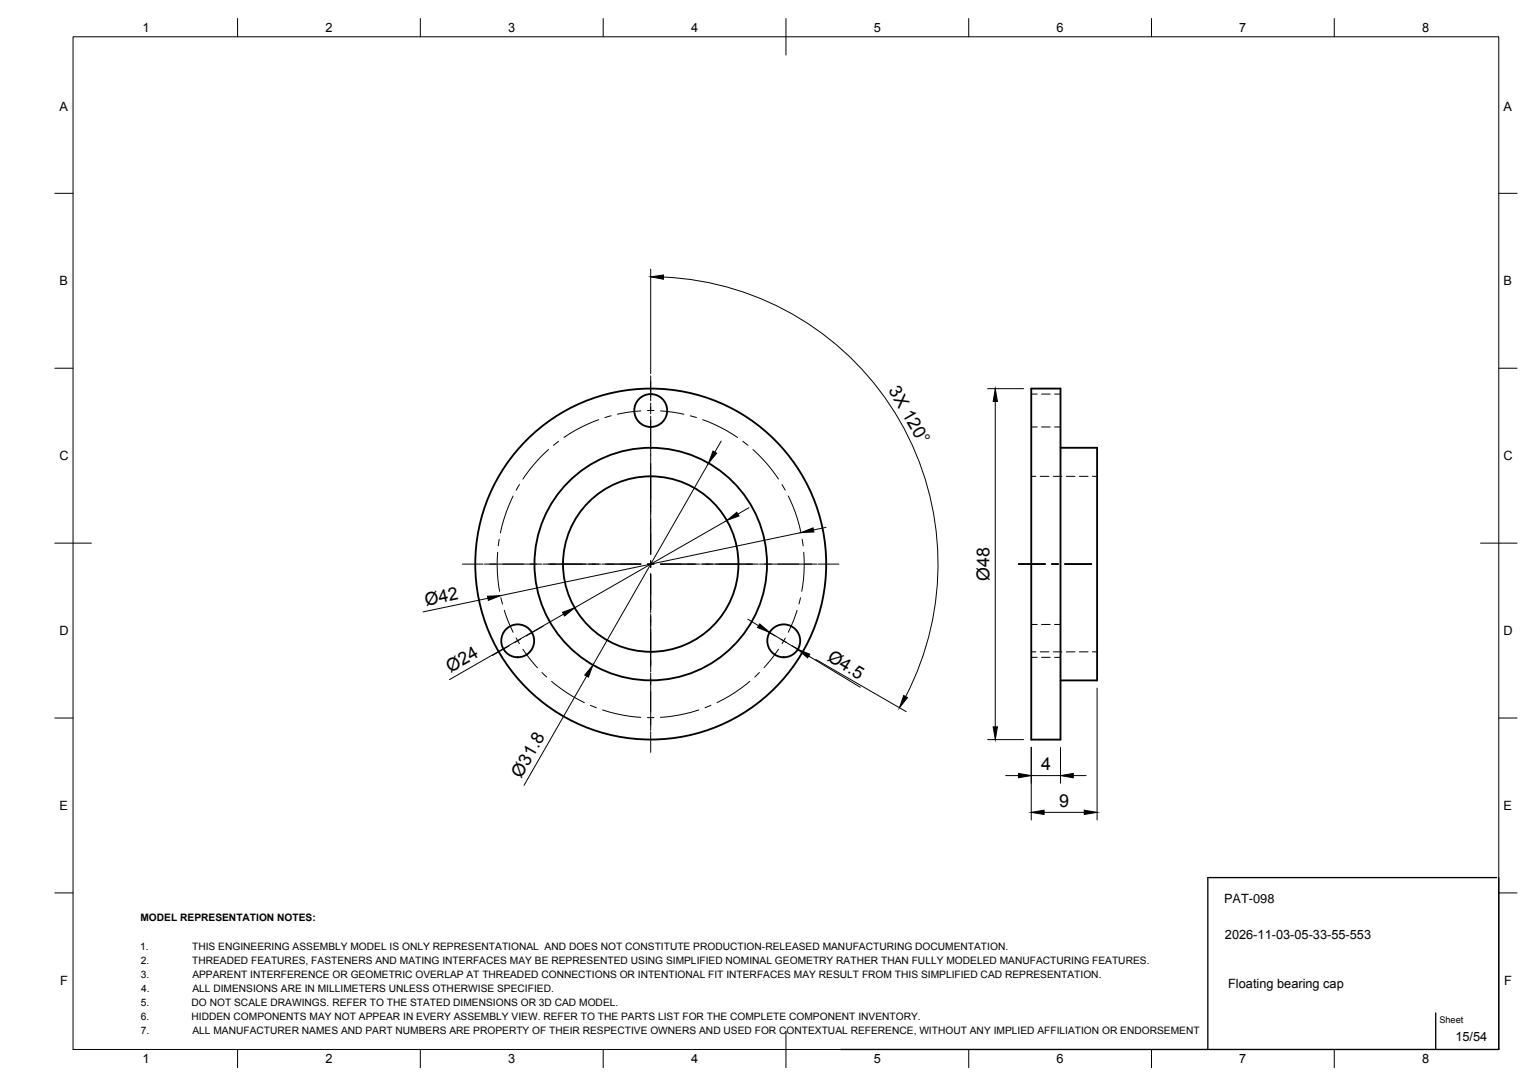
ISO-10303-21;
HEADER;
/* Generated by software containing ST-Developer
 * from STEP Tools, Inc. (www.steptools.com) 
 */

FILE_DESCRIPTION(
/* description */ ('Spring compression tester'),
/* implementation_level */ '2;1');

FILE_NAME(
/* name */ 'Floating bearing cap.step',
/* time_stamp */ '2026-10-28T03:24:11-07:00',
/* author */ (''),
/* organization */ (''),
/* preprocessor_version */ 'ST-DEVELOPER v20.2',
/* originating_system */ 'Autodesk Translation Framework v15.17.0.0',
/* authorisation */ '');

FILE_SCHEMA (('AUTOMOTIVE_DESIGN { 1 0 10303 214 3 1 1 }'));
ENDSEC;

DATA;
#10=MECHANICAL_DESIGN_GEOMETRIC_PRESENTATION_REPRESENTATION('',(#1116),#43521);
#996=SHAPE_REPRESENTATION_RELATIONSHIP('SRR','None',#43808,#1056);
#1056=ADVANCED_BREP_SHAPE_REPRESENTATION('',(#1191),#43468);
#1116=STYLED_ITEM('',(#44202),#1191);
#1191=MANIFOLD_SOLID_BREP('Body1',#18553);
#1376=FACE_BOUND('',#3547,.T.);
#1377=FACE_BOUND('',#3551,.T.);
#1378=FACE_BOUND('',#3552,.T.);
#1379=FACE_BOUND('',#3553,.T.);
#1380=FACE_BOUND('',#3554,.T.);
#1381=FACE_BOUND('',#3556,.T.);
#1382=FACE_BOUND('',#3557,.T.);
#1383=FACE_BOUND('',#3558,.T.);
#1384=FACE_BOUND('',#3559,.T.);
#1704=PLANE('',#19677);
#1705=PLANE('',#19684);
#1706=PLANE('',#19685);
#2366=FACE_OUTER_BOUND('',#3542,.T.);
#2367=FACE_OUTER_BOUND('',#3543,.T.);
#2368=FACE_OUTER_BOUND('',#3544,.T.);
#2369=FACE_OUTER_BOUND('',#3545,.T.);
#2370=FACE_OUTER_BOUND('',#3546,.T.);
#2371=FACE_OUTER_BOUND('',#3548,.T.);
#2372=FACE_OUTER_BOUND('',#3549,.T.);
#2373=FACE_OUTER_BOUND('',#3550,.T.);
#2374=FACE_OUTER_BOUND('',#3555,.T.);
#3542=EDGE_LOOP('',(#13111,#13112,#13113,#13114));
#3543=EDGE_LOOP('',(#13115,#13116,#13117,#13118));
#3544=EDGE_LOOP('',(#13119,#13120,#13121,#13122));
#3545=EDGE_LOOP('',(#13123,#13124,#13125,#13126));
#3546=EDGE_LOOP('',(#13127));
#3547=EDGE_LOOP('',(#13128));
#3548=EDGE_LOOP('',(#13129,#13130,#13131,#13132));
#3549=EDGE_LOOP('',(#13133,#13134,#13135,#13136));
#3550=EDGE_LOOP('',(#13137));
#3551=EDGE_LOOP('',(#13138));
#3552=EDGE_LOOP('',(#13139));
#3553=EDGE_LOOP('',(#13140));
#3554=EDGE_LOOP('',(#13141));
#3555=EDGE_LOOP('',(#13142));
#3556=EDGE_LOOP('',(#13143));
#3557=EDGE_LOOP('',(#13144));
#3558=EDGE_LOOP('',(#13145));
#3559=EDGE_LOOP('',(#13146));
#4883=LINE('',#27412,#6315);
#4884=LINE('',#27418,#6316);
#4885=LINE('',#27424,#6317);
#4886=LINE('',#27430,#6318);
#4887=LINE('',#27437,#6319);
#4888=LINE('',#27443,#6320);
#6315=VECTOR('',#22239,0.225);
#6316=VECTOR('',#22246,0.225);
#6317=VECTOR('',#22253,0.225);
#6318=VECTOR('',#22260,1.59);
#6319=VECTOR('',#22269,1.2);
#6320=VECTOR('',#22276,2.4);
#7640=CIRCLE('',#19666,0.225);
#7641=CIRCLE('',#19667,0.225);
#7642=CIRCLE('',#19669,0.225);
#7643=CIRCLE('',#19670,0.225);
#7644=CIRCLE('',#19672,0.225);
#7645=CIRCLE('',#19673,0.225);
#7646=CIRCLE('',#19675,1.59);
#7647=CIRCLE('',#19676,1.59);
#7648=CIRCLE('',#19678,1.2);
#7649=CIRCLE('',#19680,1.2);
#7650=CIRCLE('',#19682,2.4);
#7651=CIRCLE('',#19683,2.4);
#8434=VERTEX_POINT('',#27409);
#8435=VERTEX_POINT('',#27411);
#8436=VERTEX_POINT('',#27415);
#8437=VERTEX_POINT('',#27417);
#8438=VERTEX_POINT('',#27421);
#8439=VERTEX_POINT('',#27423);
#8440=VERTEX_POINT('',#27427);
#8441=VERTEX_POINT('',#27429);
#8442=VERTEX_POINT('',#27433);
#8443=VERTEX_POINT('',#27436);
#8444=VERTEX_POINT('',#27440);
#8445=VERTEX_POINT('',#27442);
#10220=EDGE_CURVE('',#8434,#8434,#7640,.T.);
#10221=EDGE_CURVE('',#8434,#8435,#4883,.T.);
#10222=EDGE_CURVE('',#8435,#8435,#7641,.T.);
#10223=EDGE_CURVE('',#8436,#8436,#7642,.T.);
#10224=EDGE_CURVE('',#8436,#8437,#4884,.T.);
#10225=EDGE_CURVE('',#8437,#8437,#7643,.T.);
#10226=EDGE_CURVE('',#8438,#8438,#7644,.T.);
#10227=EDGE_CURVE('',#8438,#8439,#4885,.T.);
#10228=EDGE_CURVE('',#8439,#8439,#7645,.T.);
#10229=EDGE_CURVE('',#8440,#8440,#7646,.T.);
#10230=EDGE_CURVE('',#8440,#8441,#4886,.T.);
#10231=EDGE_CURVE('',#8441,#8441,#7647,.T.);
#10232=EDGE_CURVE('',#8442,#8442,#7648,.T.);
#10233=EDGE_CURVE('',#8442,#8443,#4887,.T.);
#10234=EDGE_CURVE('',#8443,#8443,#7649,.T.);
#10235=EDGE_CURVE('',#8444,#8444,#7650,.T.);
#10236=EDGE_CURVE('',#8444,#8445,#4888,.T.);
#10237=EDGE_CURVE('',#8445,#8445,#7651,.T.);
#13111=ORIENTED_EDGE('',*,*,#10220,.F.);
#13112=ORIENTED_EDGE('',*,*,#10221,.T.);
#13113=ORIENTED_EDGE('',*,*,#10222,.F.);
#13114=ORIENTED_EDGE('',*,*,#10221,.F.);
#13115=ORIENTED_EDGE('',*,*,#10223,.F.);
#13116=ORIENTED_EDGE('',*,*,#10224,.T.);
#13117=ORIENTED_EDGE('',*,*,#10225,.F.);
#13118=ORIENTED_EDGE('',*,*,#10224,.F.);
#13119=ORIENTED_EDGE('',*,*,#10226,.F.);
#13120=ORIENTED_EDGE('',*,*,#10227,.T.);
#13121=ORIENTED_EDGE('',*,*,#10228,.F.);
#13122=ORIENTED_EDGE('',*,*,#10227,.F.);
#13123=ORIENTED_EDGE('',*,*,#10229,.F.);
#13124=ORIENTED_EDGE('',*,*,#10230,.T.);
#13125=ORIENTED_EDGE('',*,*,#10231,.F.);
#13126=ORIENTED_EDGE('',*,*,#10230,.F.);
#13127=ORIENTED_EDGE('',*,*,#10229,.T.);
#13128=ORIENTED_EDGE('',*,*,#10232,.T.);
#13129=ORIENTED_EDGE('',*,*,#10232,.F.);
#13130=ORIENTED_EDGE('',*,*,#10233,.T.);
#13131=ORIENTED_EDGE('',*,*,#10234,.T.);
#13132=ORIENTED_EDGE('',*,*,#10233,.F.);
#13133=ORIENTED_EDGE('',*,*,#10235,.F.);
#13134=ORIENTED_EDGE('',*,*,#10236,.T.);
#13135=ORIENTED_EDGE('',*,*,#10237,.T.);
#13136=ORIENTED_EDGE('',*,*,#10236,.F.);
#13137=ORIENTED_EDGE('',*,*,#10235,.T.);
#13138=ORIENTED_EDGE('',*,*,#10222,.T.);
#13139=ORIENTED_EDGE('',*,*,#10225,.T.);
#13140=ORIENTED_EDGE('',*,*,#10228,.T.);
#13141=ORIENTED_EDGE('',*,*,#10231,.T.);
#13142=ORIENTED_EDGE('',*,*,#10237,.F.);
#13143=ORIENTED_EDGE('',*,*,#10220,.T.);
#13144=ORIENTED_EDGE('',*,*,#10223,.T.);
#13145=ORIENTED_EDGE('',*,*,#10226,.T.);
#13146=ORIENTED_EDGE('',*,*,#10234,.F.);
#17186=CYLINDRICAL_SURFACE('',#19665,0.225);
#17187=CYLINDRICAL_SURFACE('',#19668,0.225);
#17188=CYLINDRICAL_SURFACE('',#19671,0.225);
#17189=CYLINDRICAL_SURFACE('',#19674,1.59);
#17190=CYLINDRICAL_SURFACE('',#19679,1.2);
#17191=CYLINDRICAL_SURFACE('',#19681,2.4);
#17690=ADVANCED_FACE('',(#2366),#17186,.F.);
#17691=ADVANCED_FACE('',(#2367),#17187,.F.);
#17692=ADVANCED_FACE('',(#2368),#17188,.F.);
#17693=ADVANCED_FACE('',(#2369),#17189,.T.);
#17694=ADVANCED_FACE('',(#2370,#1376),#1704,.T.);
#17695=ADVANCED_FACE('',(#2371),#17190,.F.);
#17696=ADVANCED_FACE('',(#2372),#17191,.T.);
#17697=ADVANCED_FACE('',(#2373,#1377,#1378,#1379,#1380),#1705,.T.);
#17698=ADVANCED_FACE('',(#2374,#1381,#1382,#1383,#1384),#1706,.F.);
#18553=CLOSED_SHELL('',(#17690,#17691,#17692,#17693,#17694,#17695,#17696,
#17697,#17698));
#19664=AXIS2_PLACEMENT_3D('',#27407,#22233,#22234);
#19665=AXIS2_PLACEMENT_3D('',#27408,#22235,#22236);
#19666=AXIS2_PLACEMENT_3D('',#27410,#22237,#22238);
#19667=AXIS2_PLACEMENT_3D('',#27413,#22240,#22241);
#19668=AXIS2_PLACEMENT_3D('',#27414,#22242,#22243);
#19669=AXIS2_PLACEMENT_3D('',#27416,#22244,#22245);
#19670=AXIS2_PLACEMENT_3D('',#27419,#22247,#22248);
#19671=AXIS2_PLACEMENT_3D('',#27420,#22249,#22250);
#19672=AXIS2_PLACEMENT_3D('',#27422,#22251,#22252);
#19673=AXIS2_PLACEMENT_3D('',#27425,#22254,#22255);
#19674=AXIS2_PLACEMENT_3D('',#27426,#22256,#22257);
#19675=AXIS2_PLACEMENT_3D('',#27428,#22258,#22259);
#19676=AXIS2_PLACEMENT_3D('',#27431,#22261,#22262);
#19677=AXIS2_PLACEMENT_3D('',#27432,#22263,#22264);
#19678=AXIS2_PLACEMENT_3D('',#27434,#22265,#22266);
#19679=AXIS2_PLACEMENT_3D('',#27435,#22267,#22268);
#19680=AXIS2_PLACEMENT_3D('',#27438,#22270,#22271);
#19681=AXIS2_PLACEMENT_3D('',#27439,#22272,#22273);
#19682=AXIS2_PLACEMENT_3D('',#27441,#22274,#22275);
#19683=AXIS2_PLACEMENT_3D('',#27444,#22277,#22278);
#19684=AXIS2_PLACEMENT_3D('',#27445,#22279,#22280);
#19685=AXIS2_PLACEMENT_3D('',#27446,#22281,#22282);
#22233=DIRECTION('axis',(0.,0.,1.));
#22234=DIRECTION('refdir',(1.,0.,0.));
#22235=DIRECTION('center_axis',(0.,0.,1.));
#22236=DIRECTION('ref_axis',(1.,0.,0.));
#22237=DIRECTION('center_axis',(0.,0.,1.));
#22238=DIRECTION('ref_axis',(1.,0.,0.));
#22239=DIRECTION('',(0.,0.,1.));
#22240=DIRECTION('center_axis',(0.,0.,-1.));
#22241=DIRECTION('ref_axis',(1.,0.,0.));
#22242=DIRECTION('center_axis',(0.,0.,1.));
#22243=DIRECTION('ref_axis',(1.,0.,0.));
#22244=DIRECTION('center_axis',(0.,0.,1.));
#22245=DIRECTION('ref_axis',(1.,0.,0.));
#22246=DIRECTION('',(0.,0.,1.));
#22247=DIRECTION('center_axis',(0.,0.,-1.));
#22248=DIRECTION('ref_axis',(1.,0.,0.));
#22249=DIRECTION('center_axis',(0.,0.,1.));
#22250=DIRECTION('ref_axis',(1.,0.,0.));
#22251=DIRECTION('center_axis',(0.,0.,1.));
#22252=DIRECTION('ref_axis',(1.,0.,0.));
#22253=DIRECTION('',(0.,0.,1.));
#22254=DIRECTION('center_axis',(0.,0.,-1.));
#22255=DIRECTION('ref_axis',(1.,0.,0.));
#22256=DIRECTION('center_axis',(0.,0.,1.));
#22257=DIRECTION('ref_axis',(1.,0.,0.));
#22258=DIRECTION('center_axis',(0.,0.,1.));
#22259=DIRECTION('ref_axis',(1.,0.,0.));
#22260=DIRECTION('',(0.,0.,-1.));
#22261=DIRECTION('center_axis',(0.,0.,-1.));
#22262=DIRECTION('ref_axis',(1.,0.,0.));
#22263=DIRECTION('center_axis',(0.,0.,1.));
#22264=DIRECTION('ref_axis',(1.,0.,0.));
#22265=DIRECTION('center_axis',(0.,0.,-1.));
#22266=DIRECTION('ref_axis',(1.,0.,0.));
#22267=DIRECTION('center_axis',(0.,0.,1.));
#22268=DIRECTION('ref_axis',(1.,0.,0.));
#22269=DIRECTION('',(0.,0.,-1.));
#22270=DIRECTION('center_axis',(0.,0.,-1.));
#22271=DIRECTION('ref_axis',(1.,0.,0.));
#22272=DIRECTION('center_axis',(0.,0.,1.));
#22273=DIRECTION('ref_axis',(1.,0.,0.));
#22274=DIRECTION('center_axis',(0.,0.,1.));
#22275=DIRECTION('ref_axis',(1.,0.,0.));
#22276=DIRECTION('',(0.,0.,-1.));
#22277=DIRECTION('center_axis',(0.,0.,1.));
#22278=DIRECTION('ref_axis',(1.,0.,0.));
#22279=DIRECTION('center_axis',(0.,0.,1.));
#22280=DIRECTION('ref_axis',(1.,0.,0.));
#22281=DIRECTION('center_axis',(0.,0.,1.));
#22282=DIRECTION('ref_axis',(1.,0.,0.));
#27407=CARTESIAN_POINT('',(0.,0.,0.));
#27408=CARTESIAN_POINT('Origin',(2.1,5.,1.5));
#27409=CARTESIAN_POINT('',(1.875,5.,1.6));
#27410=CARTESIAN_POINT('Origin',(2.1,5.,1.6));
#27411=CARTESIAN_POINT('',(1.875,5.,2.));
#27412=CARTESIAN_POINT('',(1.875,5.,1.5));
#27413=CARTESIAN_POINT('Origin',(2.1,5.,2.));
#27414=CARTESIAN_POINT('Origin',(-1.05,6.81865334794732,1.5));
#27415=CARTESIAN_POINT('',(-1.275,6.81865334794732,1.6));
#27416=CARTESIAN_POINT('Origin',(-1.05,6.81865334794732,1.6));
#27417=CARTESIAN_POINT('',(-1.275,6.81865334794732,2.));
#27418=CARTESIAN_POINT('',(-1.275,6.81865334794732,1.5));
#27419=CARTESIAN_POINT('Origin',(-1.05,6.81865334794732,2.));
#27420=CARTESIAN_POINT('Origin',(-1.05,3.18134665205268,1.5));
#27421=CARTESIAN_POINT('',(-1.275,3.18134665205268,1.6));
#27422=CARTESIAN_POINT('Origin',(-1.05,3.18134665205268,1.6));
#27423=CARTESIAN_POINT('',(-1.275,3.18134665205268,2.));
#27424=CARTESIAN_POINT('',(-1.275,3.18134665205268,1.5));
#27425=CARTESIAN_POINT('Origin',(-1.05,3.18134665205268,2.));
#27426=CARTESIAN_POINT('Origin',(0.,5.,2.));
#27427=CARTESIAN_POINT('',(-1.59,5.,2.5));
#27428=CARTESIAN_POINT('Origin',(0.,5.,2.5));
#27429=CARTESIAN_POINT('',(-1.59,5.,2.));
#27430=CARTESIAN_POINT('',(-1.59,5.,2.));
#27431=CARTESIAN_POINT('Origin',(0.,5.,2.));
#27432=CARTESIAN_POINT('Origin',(0.,5.,2.5));
#27433=CARTESIAN_POINT('',(-1.2,5.,2.5));
#27434=CARTESIAN_POINT('Origin',(0.,5.,2.5));
#27435=CARTESIAN_POINT('Origin',(0.,5.,1.6));
#27436=CARTESIAN_POINT('',(-1.2,5.,1.6));
#27437=CARTESIAN_POINT('',(-1.2,5.,1.6));
#27438=CARTESIAN_POINT('Origin',(0.,5.,1.6));
#27439=CARTESIAN_POINT('Origin',(0.,5.,1.6));
#27440=CARTESIAN_POINT('',(-2.4,5.,2.));
#27441=CARTESIAN_POINT('Origin',(0.,5.,2.));
#27442=CARTESIAN_POINT('',(-2.4,5.,1.6));
#27443=CARTESIAN_POINT('',(-2.4,5.,1.6));
#27444=CARTESIAN_POINT('Origin',(0.,5.,1.6));
#27445=CARTESIAN_POINT('Origin',(0.,5.,2.));
#27446=CARTESIAN_POINT('Origin',(0.,5.,1.6));
#43400=UNCERTAINTY_MEASURE_WITH_UNIT(LENGTH_MEASURE(0.001),#43522,
'DISTANCE_ACCURACY_VALUE',
'Maximum model space distance between geometric entities at asserted c
onnectivities');
#43453=UNCERTAINTY_MEASURE_WITH_UNIT(LENGTH_MEASURE(0.001),#43522,
'DISTANCE_ACCURACY_VALUE',
'Maximum model space distance between geometric entities at asserted c
onnectivities');
#43468=(
GEOMETRIC_REPRESENTATION_CONTEXT(3)
GLOBAL_UNCERTAINTY_ASSIGNED_CONTEXT((#43400))
GLOBAL_UNIT_ASSIGNED_CONTEXT((#43522,#43524,#43525))
REPRESENTATION_CONTEXT('','3D')
);
#43521=(
GEOMETRIC_REPRESENTATION_CONTEXT(3)
GLOBAL_UNCERTAINTY_ASSIGNED_CONTEXT((#43453))
GLOBAL_UNIT_ASSIGNED_CONTEXT((#43522,#43524,#43525))
REPRESENTATION_CONTEXT('','3D')
);
#43522=(
LENGTH_UNIT()
NAMED_UNIT(*)
SI_UNIT(.CENTI.,.METRE.)
);
#43524=(
NAMED_UNIT(*)
PLANE_ANGLE_UNIT()
SI_UNIT($,.RADIAN.)
);
#43525=(
NAMED_UNIT(*)
SI_UNIT($,.STERADIAN.)
SOLID_ANGLE_UNIT()
);
#43540=SHAPE_DEFINITION_REPRESENTATION(#43607,#43808);
#43607=PRODUCT_DEFINITION_SHAPE('',$,#43876);
#43808=SHAPE_REPRESENTATION('',(#19664),#43468);
#43861=PRODUCT_DEFINITION_CONTEXT('part definition',#44064,'design');
#43876=PRODUCT_DEFINITION('Floating bearing cap','Floating bearing cap',
#43943,#43861);
#43943=PRODUCT_DEFINITION_FORMATION('',$,#44080);
#44064=APPLICATION_CONTEXT(
'Core Data for Automotive Mechanical Design Process');
#44065=PRODUCT_CONTEXT('part definition',#44064,'mechanical');
#44080=PRODUCT('Floating bearing cap','Floating bearing cap',
'Floating bearing cap',(#44065));
#44196=COLOUR_RGB('Grey',0.48,0.52,0.57);
#44197=FILL_AREA_STYLE_COLOUR('',#44196);
#44198=FILL_AREA_STYLE('',(#44197));
#44199=SURFACE_STYLE_FILL_AREA(#44198);
#44200=SURFACE_SIDE_STYLE('',(#44199));
#44201=SURFACE_STYLE_USAGE(.BOTH.,#44200);
#44202=PRESENTATION_STYLE_ASSIGNMENT((#44201));
ENDSEC;
END-ISO-10303-21;
